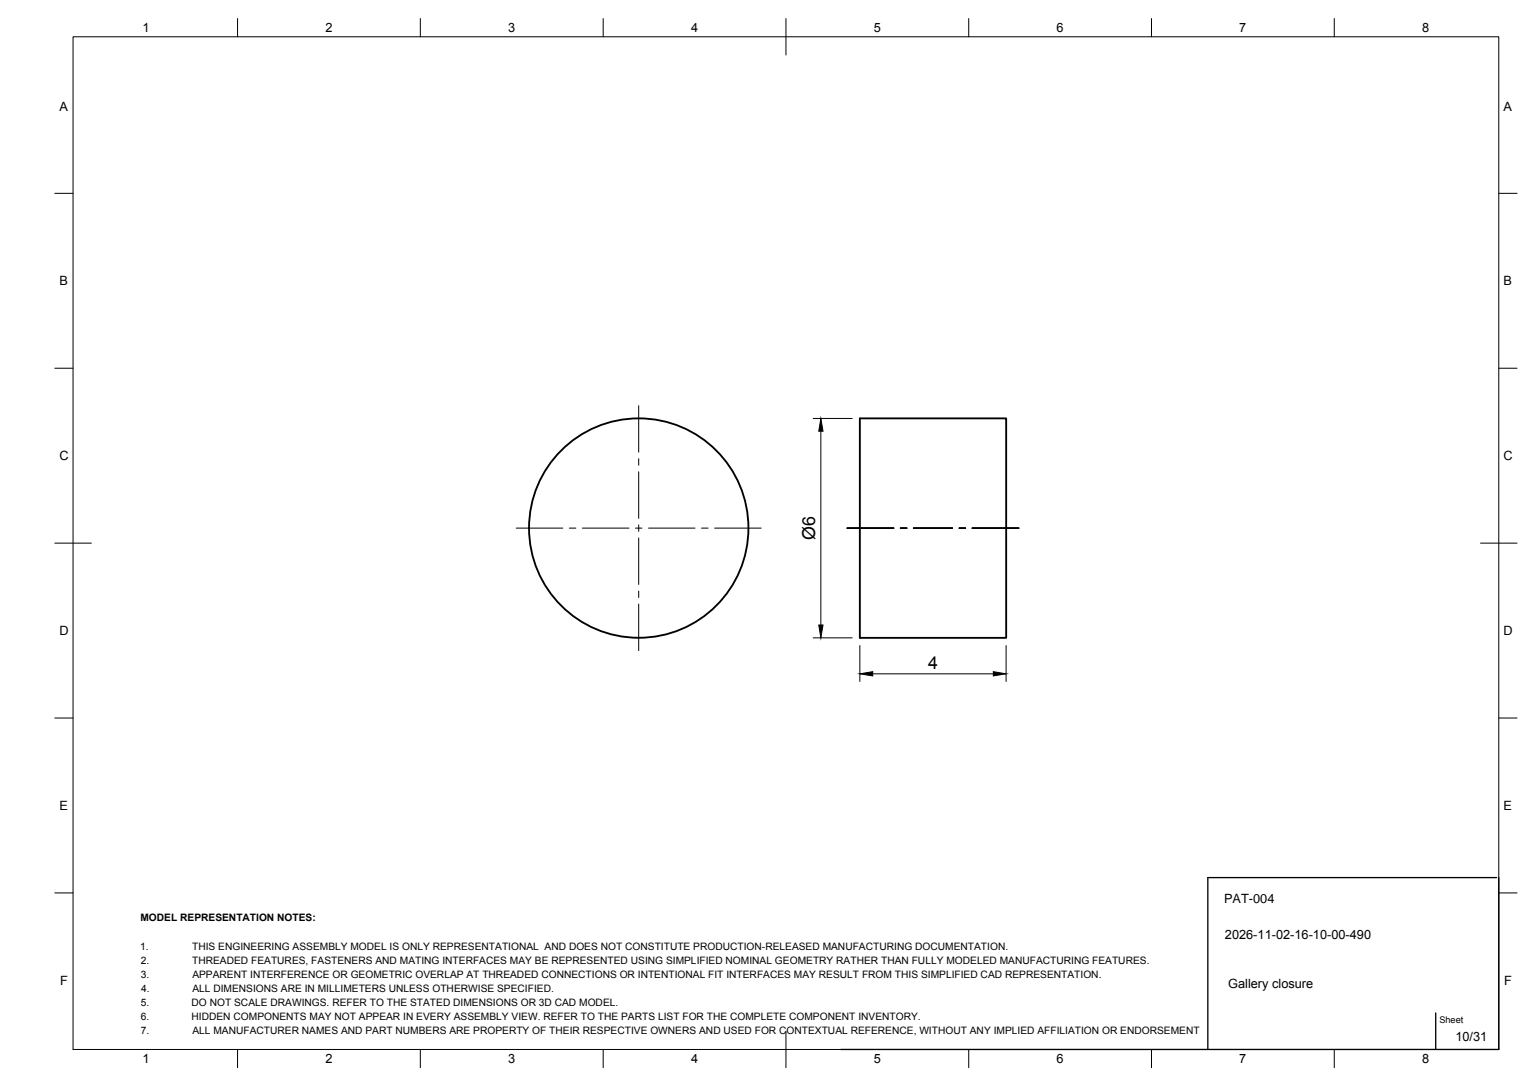
ISO-10303-21;
HEADER;
/* Generated by software containing ST-Developer
 * from STEP Tools, Inc. (www.steptools.com) 
 */

FILE_DESCRIPTION(
/* description */ ('Air blow-off nozzle station'),
/* implementation_level */ '2;1');

FILE_NAME(
/* name */ 'Gallery closure.step',
/* time_stamp */ '2026-10-27T10:53:54-07:00',
/* author */ (''),
/* organization */ (''),
/* preprocessor_version */ 'ST-DEVELOPER v20.2',
/* originating_system */ 'Autodesk Translation Framework v15.17.0.0',
/* authorisation */ '');

FILE_SCHEMA (('AUTOMOTIVE_DESIGN { 1 0 10303 214 3 1 1 }'));
ENDSEC;

DATA;
#10=MECHANICAL_DESIGN_GEOMETRIC_PRESENTATION_REPRESENTATION('',(#242),#7897);
#192=SHAPE_REPRESENTATION_RELATIONSHIP('SRR','None',#8006,#217);
#217=ADVANCED_BREP_SHAPE_REPRESENTATION('',(#267),#7873);
#242=STYLED_ITEM('',(#8213),#267);
#267=MANIFOLD_SOLID_BREP('Body1',#4291);
#413=PLANE('',#4693);
#414=PLANE('',#4694);
#598=FACE_OUTER_BOUND('',#879,.T.);
#599=FACE_OUTER_BOUND('',#880,.T.);
#600=FACE_OUTER_BOUND('',#881,.T.);
#879=EDGE_LOOP('',(#3169,#3170,#3171,#3172));
#880=EDGE_LOOP('',(#3173));
#881=EDGE_LOOP('',(#3174));
#1223=LINE('',#6919,#1577);
#1577=VECTOR('',#5363,0.300000000000001);
#1881=CIRCLE('',#4691,0.300000000000001);
#1882=CIRCLE('',#4692,0.300000000000001);
#2098=VERTEX_POINT('',#6916);
#2099=VERTEX_POINT('',#6918);
#2502=EDGE_CURVE('',#2098,#2098,#1881,.T.);
#2503=EDGE_CURVE('',#2098,#2099,#1223,.T.);
#2504=EDGE_CURVE('',#2099,#2099,#1882,.T.);
#3169=ORIENTED_EDGE('',*,*,#2502,.F.);
#3170=ORIENTED_EDGE('',*,*,#2503,.T.);
#3171=ORIENTED_EDGE('',*,*,#2504,.T.);
#3172=ORIENTED_EDGE('',*,*,#2503,.F.);
#3173=ORIENTED_EDGE('',*,*,#2502,.T.);
#3174=ORIENTED_EDGE('',*,*,#2504,.F.);
#3975=CYLINDRICAL_SURFACE('',#4690,0.300000000000001);
#4088=ADVANCED_FACE('',(#598),#3975,.T.);
#4089=ADVANCED_FACE('',(#599),#413,.T.);
#4090=ADVANCED_FACE('',(#600),#414,.F.);
#4291=CLOSED_SHELL('',(#4088,#4089,#4090));
#4689=AXIS2_PLACEMENT_3D('',#6914,#5357,#5358);
#4690=AXIS2_PLACEMENT_3D('',#6915,#5359,#5360);
#4691=AXIS2_PLACEMENT_3D('',#6917,#5361,#5362);
#4692=AXIS2_PLACEMENT_3D('',#6920,#5364,#5365);
#4693=AXIS2_PLACEMENT_3D('',#6921,#5366,#5367);
#4694=AXIS2_PLACEMENT_3D('',#6922,#5368,#5369);
#5357=DIRECTION('axis',(0.,0.,1.));
#5358=DIRECTION('refdir',(1.,0.,0.));
#5359=DIRECTION('center_axis',(1.,0.,0.));
#5360=DIRECTION('ref_axis',(0.,0.,-1.));
#5361=DIRECTION('center_axis',(1.,0.,0.));
#5362=DIRECTION('ref_axis',(0.,0.,-1.));
#5363=DIRECTION('',(-1.,0.,0.));
#5364=DIRECTION('center_axis',(1.,0.,0.));
#5365=DIRECTION('ref_axis',(0.,0.,-1.));
#5366=DIRECTION('center_axis',(1.,0.,0.));
#5367=DIRECTION('ref_axis',(0.,0.,-1.));
#5368=DIRECTION('center_axis',(1.,0.,0.));
#5369=DIRECTION('ref_axis',(0.,0.,-1.));
#6914=CARTESIAN_POINT('',(0.,0.,0.));
#6915=CARTESIAN_POINT('Origin',(-5.,0.,23.));
#6916=CARTESIAN_POINT('',(-4.6,-3.67394039744207E-17,23.3));
#6917=CARTESIAN_POINT('Origin',(-4.6,0.,23.));
#6918=CARTESIAN_POINT('',(-5.,-3.67394039744207E-17,23.3));
#6919=CARTESIAN_POINT('',(-5.,-3.67394039744207E-17,23.3));
#6920=CARTESIAN_POINT('Origin',(-5.,0.,23.));
#6921=CARTESIAN_POINT('Origin',(-4.6,0.,23.));
#6922=CARTESIAN_POINT('Origin',(-5.,0.,23.));
#7841=UNCERTAINTY_MEASURE_WITH_UNIT(LENGTH_MEASURE(0.001),#7898,
'DISTANCE_ACCURACY_VALUE',
'Maximum model space distance between geometric entities at asserted c
onnectivities');
#7865=UNCERTAINTY_MEASURE_WITH_UNIT(LENGTH_MEASURE(0.001),#7898,
'DISTANCE_ACCURACY_VALUE',
'Maximum model space distance between geometric entities at asserted c
onnectivities');
#7873=(
GEOMETRIC_REPRESENTATION_CONTEXT(3)
GLOBAL_UNCERTAINTY_ASSIGNED_CONTEXT((#7841))
GLOBAL_UNIT_ASSIGNED_CONTEXT((#7898,#7900,#7901))
REPRESENTATION_CONTEXT('','3D')
);
#7897=(
GEOMETRIC_REPRESENTATION_CONTEXT(3)
GLOBAL_UNCERTAINTY_ASSIGNED_CONTEXT((#7865))
GLOBAL_UNIT_ASSIGNED_CONTEXT((#7898,#7900,#7901))
REPRESENTATION_CONTEXT('','3D')
);
#7898=(
LENGTH_UNIT()
NAMED_UNIT(*)
SI_UNIT(.CENTI.,.METRE.)
);
#7900=(
NAMED_UNIT(*)
PLANE_ANGLE_UNIT()
SI_UNIT($,.RADIAN.)
);
#7901=(
NAMED_UNIT(*)
SI_UNIT($,.STERADIAN.)
SOLID_ANGLE_UNIT()
);
#7909=SHAPE_DEFINITION_REPRESENTATION(#7940,#8006);
#7940=PRODUCT_DEFINITION_SHAPE('',$,#8038);
#8006=SHAPE_REPRESENTATION('',(#4689),#7873);
#8030=PRODUCT_DEFINITION_CONTEXT('part definition',#8125,'design');
#8038=PRODUCT_DEFINITION('Gallery closure','Gallery closure',#8069,#8030);
#8069=PRODUCT_DEFINITION_FORMATION('',$,#8134);
#8125=APPLICATION_CONTEXT(
'Core Data for Automotive Mechanical Design Process');
#8126=PRODUCT_CONTEXT('part definition',#8125,'mechanical');
#8134=PRODUCT('Gallery closure','Gallery closure','Gallery closure',(#8126));
#8207=COLOUR_RGB('Sky Blue',0.24,0.69,0.87);
#8208=FILL_AREA_STYLE_COLOUR('',#8207);
#8209=FILL_AREA_STYLE('',(#8208));
#8210=SURFACE_STYLE_FILL_AREA(#8209);
#8211=SURFACE_SIDE_STYLE('',(#8210));
#8212=SURFACE_STYLE_USAGE(.BOTH.,#8211);
#8213=PRESENTATION_STYLE_ASSIGNMENT((#8212));
ENDSEC;
END-ISO-10303-21;
